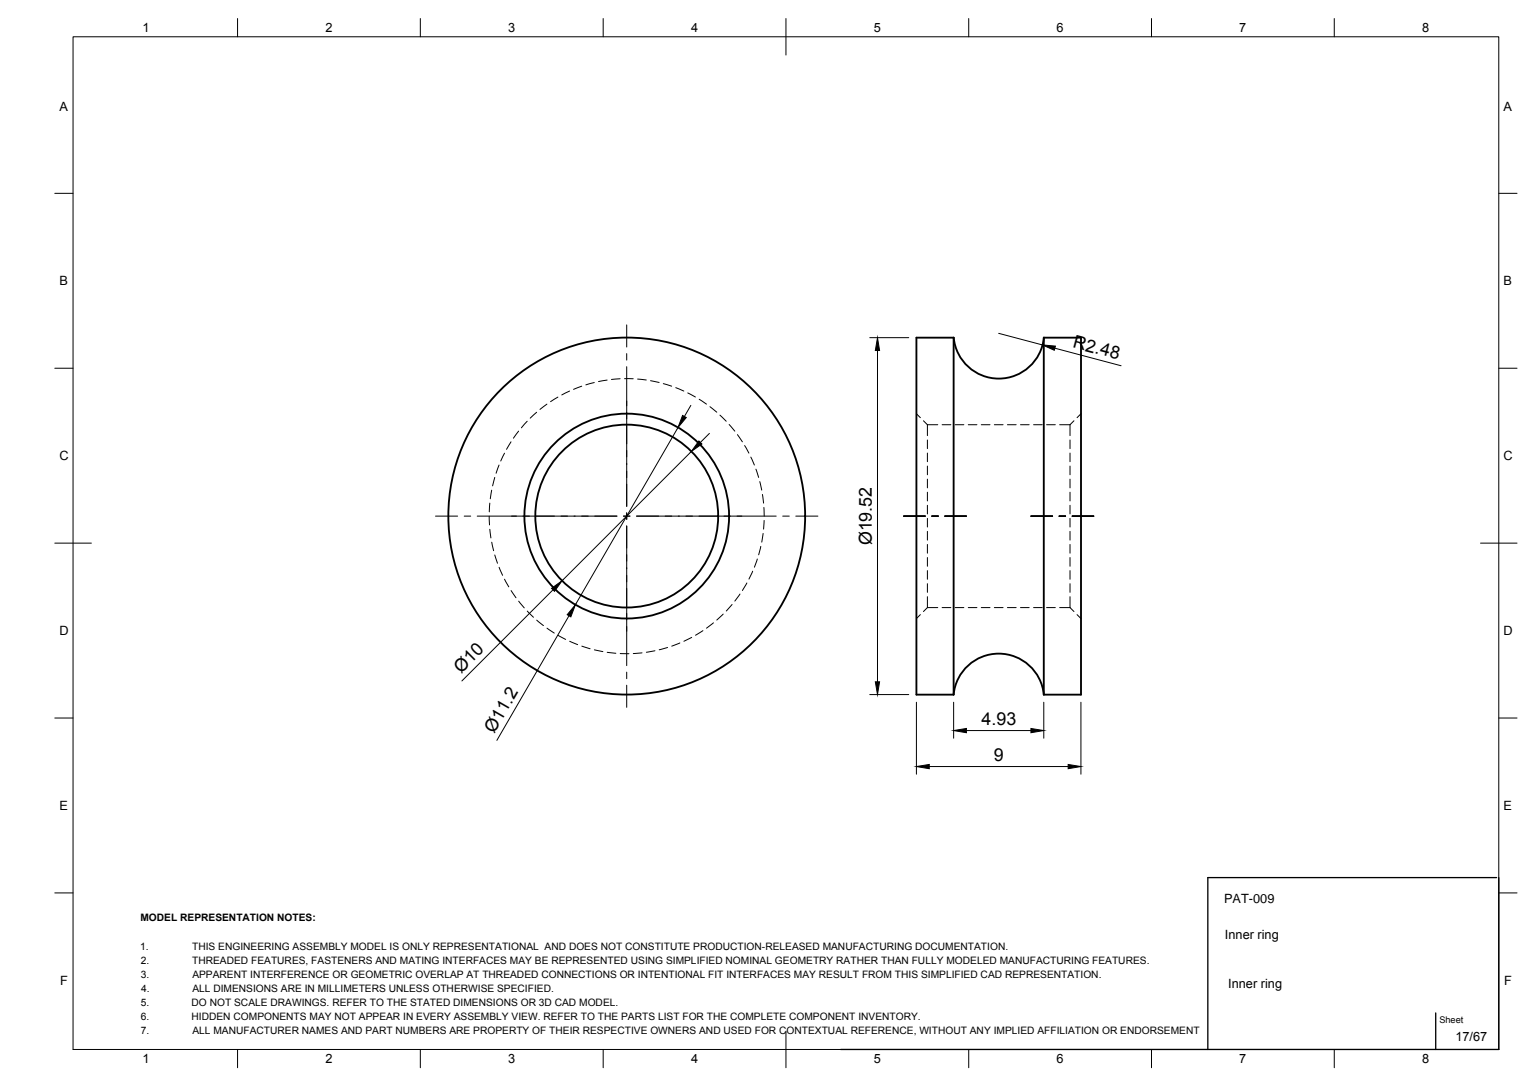
ISO-10303-21;
HEADER;
/* Generated by software containing ST-Developer
 * from STEP Tools, Inc. (www.steptools.com) 
 */

FILE_DESCRIPTION(
/* description */ ('Bell-crank linkage with push rods'),
/* implementation_level */ '2;1');

FILE_NAME(
/* name */ 'Inner ring.step',
/* time_stamp */ '2026-10-28T03:25:15-07:00',
/* author */ (''),
/* organization */ (''),
/* preprocessor_version */ 'ST-DEVELOPER v20.2',
/* originating_system */ 'Autodesk Translation Framework v15.17.0.0',
/* authorisation */ '');

FILE_SCHEMA (('AUTOMOTIVE_DESIGN { 1 0 10303 214 3 1 1 }'));
ENDSEC;

DATA;
#10=MECHANICAL_DESIGN_GEOMETRIC_PRESENTATION_REPRESENTATION('',(#614),#16678);
#431=TOROIDAL_SURFACE('',#9790,1.,0.247676);
#436=CONICAL_SURFACE('',#9801,0.53,0.785398163397448);
#437=CONICAL_SURFACE('',#9808,0.53,0.785398163397448);
#506=SHAPE_REPRESENTATION_RELATIONSHIP('SRR','None',#16923,#560);
#560=ADVANCED_BREP_SHAPE_REPRESENTATION('',(#675),#16628);
#614=STYLED_ITEM('',(#17291),#675);
#675=MANIFOLD_SOLID_BREP('Body1',#8805);
#813=FACE_BOUND('',#2025,.T.);
#814=FACE_BOUND('',#2028,.T.);
#1054=PLANE('',#9803);
#1055=PLANE('',#9806);
#1410=FACE_OUTER_BOUND('',#2020,.T.);
#1411=FACE_OUTER_BOUND('',#2021,.T.);
#1412=FACE_OUTER_BOUND('',#2022,.T.);
#1413=FACE_OUTER_BOUND('',#2023,.T.);
#1414=FACE_OUTER_BOUND('',#2024,.T.);
#1415=FACE_OUTER_BOUND('',#2026,.T.);
#1416=FACE_OUTER_BOUND('',#2027,.T.);
#1417=FACE_OUTER_BOUND('',#2029,.T.);
#2020=EDGE_LOOP('',(#6675,#6676,#6677,#6678,#6679,#6680));
#2021=EDGE_LOOP('',(#6681,#6682,#6683,#6684,#6685));
#2022=EDGE_LOOP('',(#6686,#6687,#6688,#6689));
#2023=EDGE_LOOP('',(#6690,#6691,#6692,#6693));
#2024=EDGE_LOOP('',(#6694));
#2025=EDGE_LOOP('',(#6695));
#2026=EDGE_LOOP('',(#6696,#6697,#6698,#6699,#6700));
#2027=EDGE_LOOP('',(#6701));
#2028=EDGE_LOOP('',(#6702));
#2029=EDGE_LOOP('',(#6703,#6704,#6705,#6706));
#2739=LINE('',#14489,#3288);
#2740=LINE('',#14495,#3289);
#2741=LINE('',#14499,#3290);
#2742=LINE('',#14505,#3291);
#2743=LINE('',#14510,#3292);
#3288=VECTOR('',#11523,0.976185);
#3289=VECTOR('',#11530,0.5);
#3290=VECTOR('',#11535,0.53);
#3291=VECTOR('',#11544,0.976185);
#3292=VECTOR('',#11551,0.53);
#3789=CIRCLE('',#9791,0.976185);
#3790=CIRCLE('',#9792,0.976185);
#3791=CIRCLE('',#9793,0.247676);
#3792=CIRCLE('',#9794,0.976185);
#3793=CIRCLE('',#9795,0.976185);
#3794=CIRCLE('',#9797,0.976185);
#3795=CIRCLE('',#9799,0.5);
#3796=CIRCLE('',#9800,0.5);
#3797=CIRCLE('',#9802,0.56);
#3798=CIRCLE('',#9805,0.976185);
#3799=CIRCLE('',#9807,0.56);
#4363=VERTEX_POINT('',#14478);
#4364=VERTEX_POINT('',#14479);
#4365=VERTEX_POINT('',#14482);
#4366=VERTEX_POINT('',#14484);
#4367=VERTEX_POINT('',#14488);
#4368=VERTEX_POINT('',#14492);
#4369=VERTEX_POINT('',#14494);
#4370=VERTEX_POINT('',#14498);
#4371=VERTEX_POINT('',#14503);
#4372=VERTEX_POINT('',#14507);
#5215=EDGE_CURVE('',#4363,#4364,#3789,.T.);
#5216=EDGE_CURVE('',#4364,#4363,#3790,.T.);
#5217=EDGE_CURVE('',#4364,#4365,#3791,.T.);
#5218=EDGE_CURVE('',#4366,#4365,#3792,.T.);
#5219=EDGE_CURVE('',#4365,#4366,#3793,.T.);
#5220=EDGE_CURVE('',#4366,#4367,#2739,.T.);
#5221=EDGE_CURVE('',#4367,#4367,#3794,.T.);
#5222=EDGE_CURVE('',#4368,#4368,#3795,.T.);
#5223=EDGE_CURVE('',#4368,#4369,#2740,.T.);
#5224=EDGE_CURVE('',#4369,#4369,#3796,.T.);
#5225=EDGE_CURVE('',#4369,#4370,#2741,.T.);
#5226=EDGE_CURVE('',#4370,#4370,#3797,.T.);
#5227=EDGE_CURVE('',#4371,#4371,#3798,.T.);
#5228=EDGE_CURVE('',#4371,#4363,#2742,.T.);
#5229=EDGE_CURVE('',#4372,#4372,#3799,.T.);
#5230=EDGE_CURVE('',#4372,#4368,#2743,.T.);
#6675=ORIENTED_EDGE('',*,*,#5215,.F.);
#6676=ORIENTED_EDGE('',*,*,#5216,.F.);
#6677=ORIENTED_EDGE('',*,*,#5217,.T.);
#6678=ORIENTED_EDGE('',*,*,#5218,.F.);
#6679=ORIENTED_EDGE('',*,*,#5219,.F.);
#6680=ORIENTED_EDGE('',*,*,#5217,.F.);
#6681=ORIENTED_EDGE('',*,*,#5218,.T.);
#6682=ORIENTED_EDGE('',*,*,#5219,.T.);
#6683=ORIENTED_EDGE('',*,*,#5220,.T.);
#6684=ORIENTED_EDGE('',*,*,#5221,.T.);
#6685=ORIENTED_EDGE('',*,*,#5220,.F.);
#6686=ORIENTED_EDGE('',*,*,#5222,.T.);
#6687=ORIENTED_EDGE('',*,*,#5223,.T.);
#6688=ORIENTED_EDGE('',*,*,#5224,.F.);
#6689=ORIENTED_EDGE('',*,*,#5223,.F.);
#6690=ORIENTED_EDGE('',*,*,#5224,.T.);
#6691=ORIENTED_EDGE('',*,*,#5225,.T.);
#6692=ORIENTED_EDGE('',*,*,#5226,.F.);
#6693=ORIENTED_EDGE('',*,*,#5225,.F.);
#6694=ORIENTED_EDGE('',*,*,#5221,.F.);
#6695=ORIENTED_EDGE('',*,*,#5226,.T.);
#6696=ORIENTED_EDGE('',*,*,#5227,.F.);
#6697=ORIENTED_EDGE('',*,*,#5228,.T.);
#6698=ORIENTED_EDGE('',*,*,#5215,.T.);
#6699=ORIENTED_EDGE('',*,*,#5216,.T.);
#6700=ORIENTED_EDGE('',*,*,#5228,.F.);
#6701=ORIENTED_EDGE('',*,*,#5227,.T.);
#6702=ORIENTED_EDGE('',*,*,#5229,.F.);
#6703=ORIENTED_EDGE('',*,*,#5229,.T.);
#6704=ORIENTED_EDGE('',*,*,#5230,.T.);
#6705=ORIENTED_EDGE('',*,*,#5222,.F.);
#6706=ORIENTED_EDGE('',*,*,#5230,.F.);
#8139=CYLINDRICAL_SURFACE('',#9796,0.976185);
#8140=CYLINDRICAL_SURFACE('',#9798,0.5);
#8141=CYLINDRICAL_SURFACE('',#9804,0.976185);
#8435=ADVANCED_FACE('',(#1410),#431,.F.);
#8436=ADVANCED_FACE('',(#1411),#8139,.T.);
#8437=ADVANCED_FACE('',(#1412),#8140,.F.);
#8438=ADVANCED_FACE('',(#1413),#436,.F.);
#8439=ADVANCED_FACE('',(#1414,#813),#1054,.T.);
#8440=ADVANCED_FACE('',(#1415),#8141,.T.);
#8441=ADVANCED_FACE('',(#1416,#814),#1055,.T.);
#8442=ADVANCED_FACE('',(#1417),#437,.F.);
#8805=CLOSED_SHELL('',(#8435,#8436,#8437,#8438,#8439,#8440,#8441,#8442));
#9789=AXIS2_PLACEMENT_3D('',#14476,#11507,#11508);
#9790=AXIS2_PLACEMENT_3D('',#14477,#11509,#11510);
#9791=AXIS2_PLACEMENT_3D('',#14480,#11511,#11512);
#9792=AXIS2_PLACEMENT_3D('',#14481,#11513,#11514);
#9793=AXIS2_PLACEMENT_3D('',#14483,#11515,#11516);
#9794=AXIS2_PLACEMENT_3D('',#14485,#11517,#11518);
#9795=AXIS2_PLACEMENT_3D('',#14486,#11519,#11520);
#9796=AXIS2_PLACEMENT_3D('',#14487,#11521,#11522);
#9797=AXIS2_PLACEMENT_3D('',#14490,#11524,#11525);
#9798=AXIS2_PLACEMENT_3D('',#14491,#11526,#11527);
#9799=AXIS2_PLACEMENT_3D('',#14493,#11528,#11529);
#9800=AXIS2_PLACEMENT_3D('',#14496,#11531,#11532);
#9801=AXIS2_PLACEMENT_3D('',#14497,#11533,#11534);
#9802=AXIS2_PLACEMENT_3D('',#14500,#11536,#11537);
#9803=AXIS2_PLACEMENT_3D('',#14501,#11538,#11539);
#9804=AXIS2_PLACEMENT_3D('',#14502,#11540,#11541);
#9805=AXIS2_PLACEMENT_3D('',#14504,#11542,#11543);
#9806=AXIS2_PLACEMENT_3D('',#14506,#11545,#11546);
#9807=AXIS2_PLACEMENT_3D('',#14508,#11547,#11548);
#9808=AXIS2_PLACEMENT_3D('',#14509,#11549,#11550);
#11507=DIRECTION('axis',(0.,0.,1.));
#11508=DIRECTION('refdir',(1.,0.,0.));
#11509=DIRECTION('center_axis',(0.,-1.,0.));
#11510=DIRECTION('ref_axis',(0.,0.,-1.));
#11511=DIRECTION('center_axis',(0.,-1.,0.));
#11512=DIRECTION('ref_axis',(1.,0.,0.));
#11513=DIRECTION('center_axis',(0.,-1.,0.));
#11514=DIRECTION('ref_axis',(1.,0.,0.));
#11515=DIRECTION('center_axis',(1.,0.,1.22464679914735E-16));
#11516=DIRECTION('ref_axis',(-1.22464679914735E-16,0.,1.));
#11517=DIRECTION('center_axis',(0.,1.,0.));
#11518=DIRECTION('ref_axis',(1.,0.,0.));
#11519=DIRECTION('center_axis',(0.,1.,0.));
#11520=DIRECTION('ref_axis',(1.,0.,0.));
#11521=DIRECTION('center_axis',(0.,-1.,0.));
#11522=DIRECTION('ref_axis',(1.,0.,0.));
#11523=DIRECTION('',(0.,1.,0.));
#11524=DIRECTION('center_axis',(0.,-1.,0.));
#11525=DIRECTION('ref_axis',(1.,0.,0.));
#11526=DIRECTION('center_axis',(0.,-1.,0.));
#11527=DIRECTION('ref_axis',(1.,0.,0.));
#11528=DIRECTION('center_axis',(0.,-1.,0.));
#11529=DIRECTION('ref_axis',(1.,0.,0.));
#11530=DIRECTION('',(0.,1.,0.));
#11531=DIRECTION('center_axis',(0.,-1.,0.));
#11532=DIRECTION('ref_axis',(1.,0.,0.));
#11533=DIRECTION('center_axis',(0.,1.,0.));
#11534=DIRECTION('ref_axis',(1.,0.,0.));
#11535=DIRECTION('',(-0.707106781186547,0.707106781186548,-8.65956056235493E-17));
#11536=DIRECTION('center_axis',(0.,-1.,0.));
#11537=DIRECTION('ref_axis',(1.,0.,0.));
#11538=DIRECTION('center_axis',(0.,1.,0.));
#11539=DIRECTION('ref_axis',(0.,0.,1.));
#11540=DIRECTION('center_axis',(0.,-1.,0.));
#11541=DIRECTION('ref_axis',(1.,0.,0.));
#11542=DIRECTION('center_axis',(0.,-1.,0.));
#11543=DIRECTION('ref_axis',(1.,0.,0.));
#11544=DIRECTION('',(0.,1.,0.));
#11545=DIRECTION('center_axis',(0.,-1.,0.));
#11546=DIRECTION('ref_axis',(0.,0.,-1.));
#11547=DIRECTION('center_axis',(0.,-1.,0.));
#11548=DIRECTION('ref_axis',(1.,0.,0.));
#11549=DIRECTION('center_axis',(0.,-1.,0.));
#11550=DIRECTION('ref_axis',(1.,0.,0.));
#11551=DIRECTION('',(0.707106781186547,0.707106781186548,8.65956056235493E-17));
#14476=CARTESIAN_POINT('',(0.,0.,0.));
#14477=CARTESIAN_POINT('Origin',(0.,0.,0.));
#14478=CARTESIAN_POINT('',(-0.976185,-0.246528389340863,-1.19548183562566E-16));
#14479=CARTESIAN_POINT('',(-1.19548183562566E-16,-0.246528389340863,0.976185));
#14480=CARTESIAN_POINT('Origin',(0.,-0.246528389340863,0.));
#14481=CARTESIAN_POINT('Origin',(0.,-0.246528389340863,0.));
#14482=CARTESIAN_POINT('',(-1.19548183562566E-16,0.246528389340863,0.976185));
#14483=CARTESIAN_POINT('Origin',(-1.22464679914735E-16,0.,1.));
#14484=CARTESIAN_POINT('',(-0.976185,0.246528389340863,1.19548183562566E-16));
#14485=CARTESIAN_POINT('Origin',(0.,0.246528389340863,0.));
#14486=CARTESIAN_POINT('Origin',(0.,0.246528389340863,0.));
#14487=CARTESIAN_POINT('Origin',(0.,0.,0.));
#14488=CARTESIAN_POINT('',(-0.976185,0.45,-1.19548183562566E-16));
#14489=CARTESIAN_POINT('',(-0.976185,0.,-1.19548183562566E-16));
#14490=CARTESIAN_POINT('Origin',(0.,0.45,0.));
#14491=CARTESIAN_POINT('Origin',(0.,0.,0.));
#14492=CARTESIAN_POINT('',(-0.5,-0.39,-6.12323399573677E-17));
#14493=CARTESIAN_POINT('Origin',(0.,-0.39,0.));
#14494=CARTESIAN_POINT('',(-0.5,0.39,-6.12323399573677E-17));
#14495=CARTESIAN_POINT('',(-0.5,0.,-6.12323399573677E-17));
#14496=CARTESIAN_POINT('Origin',(0.,0.39,0.));
#14497=CARTESIAN_POINT('Origin',(0.,0.42,0.));
#14498=CARTESIAN_POINT('',(-0.56,0.45,-6.85802207522518E-17));
#14499=CARTESIAN_POINT('',(-0.53,0.42,-6.49062803548097E-17));
#14500=CARTESIAN_POINT('Origin',(0.,0.45,0.));
#14501=CARTESIAN_POINT('Origin',(0.976185,0.45,0.));
#14502=CARTESIAN_POINT('Origin',(0.,0.,0.));
#14503=CARTESIAN_POINT('',(-0.976185,-0.45,-1.19548183562566E-16));
#14504=CARTESIAN_POINT('Origin',(0.,-0.45,0.));
#14505=CARTESIAN_POINT('',(-0.976185,0.,-1.19548183562566E-16));
#14506=CARTESIAN_POINT('Origin',(0.56,-0.45,0.));
#14507=CARTESIAN_POINT('',(-0.56,-0.45,-6.85802207522518E-17));
#14508=CARTESIAN_POINT('Origin',(0.,-0.45,0.));
#14509=CARTESIAN_POINT('Origin',(0.,-0.42,0.));
#14510=CARTESIAN_POINT('',(-0.53,-0.42,-6.49062803548097E-17));
#16564=UNCERTAINTY_MEASURE_WITH_UNIT(LENGTH_MEASURE(0.001),#16679,
'DISTANCE_ACCURACY_VALUE',
'Maximum model space distance between geometric entities at asserted c
onnectivities');
#16614=UNCERTAINTY_MEASURE_WITH_UNIT(LENGTH_MEASURE(0.001),#16679,
'DISTANCE_ACCURACY_VALUE',
'Maximum model space distance between geometric entities at asserted c
onnectivities');
#16628=(
GEOMETRIC_REPRESENTATION_CONTEXT(3)
GLOBAL_UNCERTAINTY_ASSIGNED_CONTEXT((#16564))
GLOBAL_UNIT_ASSIGNED_CONTEXT((#16679,#16681,#16682))
REPRESENTATION_CONTEXT('','3D')
);
#16678=(
GEOMETRIC_REPRESENTATION_CONTEXT(3)
GLOBAL_UNCERTAINTY_ASSIGNED_CONTEXT((#16614))
GLOBAL_UNIT_ASSIGNED_CONTEXT((#16679,#16681,#16682))
REPRESENTATION_CONTEXT('','3D')
);
#16679=(
LENGTH_UNIT()
NAMED_UNIT(*)
SI_UNIT(.CENTI.,.METRE.)
);
#16681=(
NAMED_UNIT(*)
PLANE_ANGLE_UNIT()
SI_UNIT($,.RADIAN.)
);
#16682=(
NAMED_UNIT(*)
SI_UNIT($,.STERADIAN.)
SOLID_ANGLE_UNIT()
);
#16696=SHAPE_DEFINITION_REPRESENTATION(#16759,#16923);
#16759=PRODUCT_DEFINITION_SHAPE('',$,#16987);
#16923=SHAPE_REPRESENTATION('',(#9789),#16628);
#16973=PRODUCT_DEFINITION_CONTEXT('part definition',#17164,'design');
#16987=PRODUCT_DEFINITION('Inner ring','Inner ring',#17050,#16973);
#17050=PRODUCT_DEFINITION_FORMATION('',$,#17179);
#17164=APPLICATION_CONTEXT(
'Core Data for Automotive Mechanical Design Process');
#17165=PRODUCT_CONTEXT('part definition',#17164,'mechanical');
#17179=PRODUCT('Inner ring','Inner ring','Inner ring',(#17165));
#17285=COLOUR_RGB('Grey',0.48,0.52,0.57);
#17286=FILL_AREA_STYLE_COLOUR('',#17285);
#17287=FILL_AREA_STYLE('',(#17286));
#17288=SURFACE_STYLE_FILL_AREA(#17287);
#17289=SURFACE_SIDE_STYLE('',(#17288));
#17290=SURFACE_STYLE_USAGE(.BOTH.,#17289);
#17291=PRESENTATION_STYLE_ASSIGNMENT((#17290));
ENDSEC;
END-ISO-10303-21;
